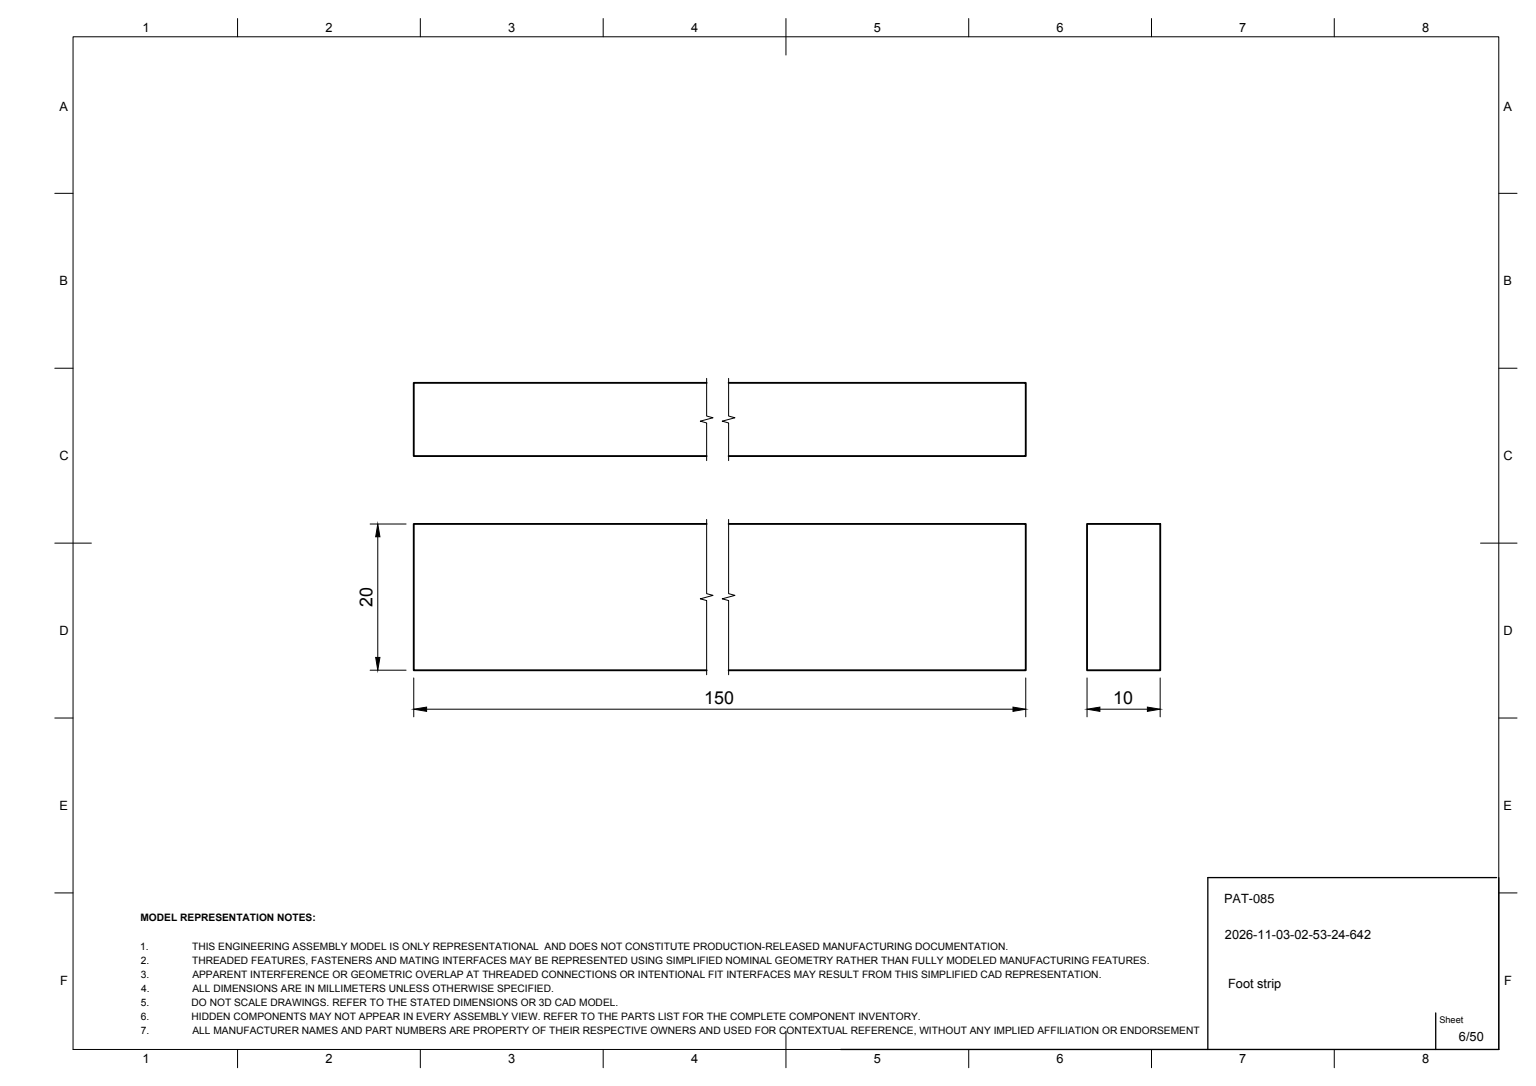
ISO-10303-21;
HEADER;
/* Generated by software containing ST-Developer
 * from STEP Tools, Inc. (www.steptools.com) 
 */

FILE_DESCRIPTION(
/* description */ ('Rack and pinion manual slide'),
/* implementation_level */ '2;1');

FILE_NAME(
/* name */ 'Foot strip.step',
/* time_stamp */ '2026-10-28T03:22:49-07:00',
/* author */ (''),
/* organization */ (''),
/* preprocessor_version */ 'ST-DEVELOPER v20.2',
/* originating_system */ 'Autodesk Translation Framework v15.17.0.0',
/* authorisation */ '');

FILE_SCHEMA (('AUTOMOTIVE_DESIGN { 1 0 10303 214 3 1 1 }'));
ENDSEC;

DATA;
#10=MECHANICAL_DESIGN_GEOMETRIC_PRESENTATION_REPRESENTATION('',(#733),#34851);
#641=SHAPE_REPRESENTATION_RELATIONSHIP('SRR','None',#35076,#687);
#687=ADVANCED_BREP_SHAPE_REPRESENTATION('',(#786),#34801);
#733=STYLED_ITEM('',(#35397),#786);
#786=MANIFOLD_SOLID_BREP('Body1',#13753);
#1050=PLANE('',#14339);
#1051=PLANE('',#14340);
#1052=PLANE('',#14341);
#1053=PLANE('',#14342);
#1054=PLANE('',#14343);
#1055=PLANE('',#14344);
#1545=FACE_OUTER_BOUND('',#2292,.T.);
#1546=FACE_OUTER_BOUND('',#2293,.T.);
#1547=FACE_OUTER_BOUND('',#2294,.T.);
#1548=FACE_OUTER_BOUND('',#2295,.T.);
#1549=FACE_OUTER_BOUND('',#2296,.T.);
#1550=FACE_OUTER_BOUND('',#2297,.T.);
#2292=EDGE_LOOP('',(#9282,#9283,#9284,#9285));
#2293=EDGE_LOOP('',(#9286,#9287,#9288,#9289));
#2294=EDGE_LOOP('',(#9290,#9291,#9292,#9293));
#2295=EDGE_LOOP('',(#9294,#9295,#9296,#9297));
#2296=EDGE_LOOP('',(#9298,#9299,#9300,#9301));
#2297=EDGE_LOOP('',(#9302,#9303,#9304,#9305));
#3240=LINE('',#19514,#4531);
#3241=LINE('',#19516,#4532);
#3242=LINE('',#19518,#4533);
#3243=LINE('',#19519,#4534);
#3244=LINE('',#19522,#4535);
#3245=LINE('',#19524,#4536);
#3246=LINE('',#19525,#4537);
#3247=LINE('',#19528,#4538);
#3248=LINE('',#19530,#4539);
#3249=LINE('',#19531,#4540);
#3250=LINE('',#19533,#4541);
#3251=LINE('',#19534,#4542);
#4531=VECTOR('',#15662,1.);
#4532=VECTOR('',#15663,1.);
#4533=VECTOR('',#15664,1.);
#4534=VECTOR('',#15665,1.);
#4535=VECTOR('',#15668,1.);
#4536=VECTOR('',#15669,1.);
#4537=VECTOR('',#15670,1.);
#4538=VECTOR('',#15673,1.);
#4539=VECTOR('',#15674,1.);
#4540=VECTOR('',#15675,1.);
#4541=VECTOR('',#15678,1.);
#4542=VECTOR('',#15679,1.);
#6240=VERTEX_POINT('',#19512);
#6241=VERTEX_POINT('',#19513);
#6242=VERTEX_POINT('',#19515);
#6243=VERTEX_POINT('',#19517);
#6244=VERTEX_POINT('',#19521);
#6245=VERTEX_POINT('',#19523);
#6246=VERTEX_POINT('',#19527);
#6247=VERTEX_POINT('',#19529);
#7453=EDGE_CURVE('',#6240,#6241,#3240,.T.);
#7454=EDGE_CURVE('',#6241,#6242,#3241,.T.);
#7455=EDGE_CURVE('',#6243,#6242,#3242,.T.);
#7456=EDGE_CURVE('',#6240,#6243,#3243,.T.);
#7457=EDGE_CURVE('',#6244,#6240,#3244,.T.);
#7458=EDGE_CURVE('',#6245,#6243,#3245,.T.);
#7459=EDGE_CURVE('',#6244,#6245,#3246,.T.);
#7460=EDGE_CURVE('',#6246,#6244,#3247,.T.);
#7461=EDGE_CURVE('',#6247,#6245,#3248,.T.);
#7462=EDGE_CURVE('',#6246,#6247,#3249,.T.);
#7463=EDGE_CURVE('',#6241,#6246,#3250,.T.);
#7464=EDGE_CURVE('',#6242,#6247,#3251,.T.);
#9282=ORIENTED_EDGE('',*,*,#7453,.T.);
#9283=ORIENTED_EDGE('',*,*,#7454,.T.);
#9284=ORIENTED_EDGE('',*,*,#7455,.F.);
#9285=ORIENTED_EDGE('',*,*,#7456,.F.);
#9286=ORIENTED_EDGE('',*,*,#7457,.T.);
#9287=ORIENTED_EDGE('',*,*,#7456,.T.);
#9288=ORIENTED_EDGE('',*,*,#7458,.F.);
#9289=ORIENTED_EDGE('',*,*,#7459,.F.);
#9290=ORIENTED_EDGE('',*,*,#7460,.T.);
#9291=ORIENTED_EDGE('',*,*,#7459,.T.);
#9292=ORIENTED_EDGE('',*,*,#7461,.F.);
#9293=ORIENTED_EDGE('',*,*,#7462,.F.);
#9294=ORIENTED_EDGE('',*,*,#7463,.T.);
#9295=ORIENTED_EDGE('',*,*,#7462,.T.);
#9296=ORIENTED_EDGE('',*,*,#7464,.F.);
#9297=ORIENTED_EDGE('',*,*,#7454,.F.);
#9298=ORIENTED_EDGE('',*,*,#7464,.T.);
#9299=ORIENTED_EDGE('',*,*,#7461,.T.);
#9300=ORIENTED_EDGE('',*,*,#7458,.T.);
#9301=ORIENTED_EDGE('',*,*,#7455,.T.);
#9302=ORIENTED_EDGE('',*,*,#7463,.F.);
#9303=ORIENTED_EDGE('',*,*,#7453,.F.);
#9304=ORIENTED_EDGE('',*,*,#7457,.F.);
#9305=ORIENTED_EDGE('',*,*,#7460,.F.);
#13023=ADVANCED_FACE('',(#1545),#1050,.T.);
#13024=ADVANCED_FACE('',(#1546),#1051,.T.);
#13025=ADVANCED_FACE('',(#1547),#1052,.T.);
#13026=ADVANCED_FACE('',(#1548),#1053,.T.);
#13027=ADVANCED_FACE('',(#1549),#1054,.T.);
#13028=ADVANCED_FACE('',(#1550),#1055,.F.);
#13753=CLOSED_SHELL('',(#13023,#13024,#13025,#13026,#13027,#13028));
#14338=AXIS2_PLACEMENT_3D('',#19510,#15658,#15659);
#14339=AXIS2_PLACEMENT_3D('',#19511,#15660,#15661);
#14340=AXIS2_PLACEMENT_3D('',#19520,#15666,#15667);
#14341=AXIS2_PLACEMENT_3D('',#19526,#15671,#15672);
#14342=AXIS2_PLACEMENT_3D('',#19532,#15676,#15677);
#14343=AXIS2_PLACEMENT_3D('',#19535,#15680,#15681);
#14344=AXIS2_PLACEMENT_3D('',#19536,#15682,#15683);
#15658=DIRECTION('axis',(0.,0.,1.));
#15659=DIRECTION('refdir',(1.,0.,0.));
#15660=DIRECTION('center_axis',(0.,1.,0.));
#15661=DIRECTION('ref_axis',(-1.,0.,0.));
#15662=DIRECTION('',(-1.,0.,0.));
#15663=DIRECTION('',(0.,0.,1.));
#15664=DIRECTION('',(-1.,0.,0.));
#15665=DIRECTION('',(0.,0.,1.));
#15666=DIRECTION('center_axis',(1.,0.,0.));
#15667=DIRECTION('ref_axis',(0.,1.,0.));
#15668=DIRECTION('',(0.,1.,0.));
#15669=DIRECTION('',(0.,1.,0.));
#15670=DIRECTION('',(0.,0.,1.));
#15671=DIRECTION('center_axis',(0.,-1.,0.));
#15672=DIRECTION('ref_axis',(1.,0.,0.));
#15673=DIRECTION('',(1.,0.,0.));
#15674=DIRECTION('',(1.,0.,0.));
#15675=DIRECTION('',(0.,0.,1.));
#15676=DIRECTION('center_axis',(-1.,0.,0.));
#15677=DIRECTION('ref_axis',(0.,-1.,0.));
#15678=DIRECTION('',(0.,-1.,0.));
#15679=DIRECTION('',(0.,-1.,0.));
#15680=DIRECTION('center_axis',(0.,0.,1.));
#15681=DIRECTION('ref_axis',(1.,0.,0.));
#15682=DIRECTION('center_axis',(0.,0.,1.));
#15683=DIRECTION('ref_axis',(1.,0.,0.));
#19510=CARTESIAN_POINT('',(0.,0.,0.));
#19511=CARTESIAN_POINT('Origin',(-4.,7.5,-1.));
#19512=CARTESIAN_POINT('',(-4.,7.5,-1.));
#19513=CARTESIAN_POINT('',(-6.,7.5,-1.));
#19514=CARTESIAN_POINT('',(-4.,7.5,-1.));
#19515=CARTESIAN_POINT('',(-6.,7.5,0.));
#19516=CARTESIAN_POINT('',(-6.,7.5,-1.));
#19517=CARTESIAN_POINT('',(-4.,7.5,0.));
#19518=CARTESIAN_POINT('',(-4.,7.5,0.));
#19519=CARTESIAN_POINT('',(-4.,7.5,-1.));
#19520=CARTESIAN_POINT('Origin',(-4.,-7.5,-1.));
#19521=CARTESIAN_POINT('',(-4.,-7.5,-1.));
#19522=CARTESIAN_POINT('',(-4.,-7.5,-1.));
#19523=CARTESIAN_POINT('',(-4.,-7.5,0.));
#19524=CARTESIAN_POINT('',(-4.,-7.5,0.));
#19525=CARTESIAN_POINT('',(-4.,-7.5,-1.));
#19526=CARTESIAN_POINT('Origin',(-6.,-7.5,-1.));
#19527=CARTESIAN_POINT('',(-6.,-7.5,-1.));
#19528=CARTESIAN_POINT('',(-6.,-7.5,-1.));
#19529=CARTESIAN_POINT('',(-6.,-7.5,0.));
#19530=CARTESIAN_POINT('',(-6.,-7.5,0.));
#19531=CARTESIAN_POINT('',(-6.,-7.5,-1.));
#19532=CARTESIAN_POINT('Origin',(-6.,7.5,-1.));
#19533=CARTESIAN_POINT('',(-6.,7.5,-1.));
#19534=CARTESIAN_POINT('',(-6.,7.5,0.));
#19535=CARTESIAN_POINT('Origin',(-5.,0.,0.));
#19536=CARTESIAN_POINT('Origin',(-5.,0.,-1.));
#34747=UNCERTAINTY_MEASURE_WITH_UNIT(LENGTH_MEASURE(0.001),#34852,
'DISTANCE_ACCURACY_VALUE',
'Maximum model space distance between geometric entities at asserted c
onnectivities');
#34797=UNCERTAINTY_MEASURE_WITH_UNIT(LENGTH_MEASURE(0.001),#34852,
'DISTANCE_ACCURACY_VALUE',
'Maximum model space distance between geometric entities at asserted c
onnectivities');
#34801=(
GEOMETRIC_REPRESENTATION_CONTEXT(3)
GLOBAL_UNCERTAINTY_ASSIGNED_CONTEXT((#34747))
GLOBAL_UNIT_ASSIGNED_CONTEXT((#34852,#34854,#34855))
REPRESENTATION_CONTEXT('','3D')
);
#34851=(
GEOMETRIC_REPRESENTATION_CONTEXT(3)
GLOBAL_UNCERTAINTY_ASSIGNED_CONTEXT((#34797))
GLOBAL_UNIT_ASSIGNED_CONTEXT((#34852,#34854,#34855))
REPRESENTATION_CONTEXT('','3D')
);
#34852=(
LENGTH_UNIT()
NAMED_UNIT(*)
SI_UNIT(.CENTI.,.METRE.)
);
#34854=(
NAMED_UNIT(*)
PLANE_ANGLE_UNIT()
SI_UNIT($,.RADIAN.)
);
#34855=(
NAMED_UNIT(*)
SI_UNIT($,.STERADIAN.)
SOLID_ANGLE_UNIT()
);
#34859=SHAPE_DEFINITION_REPRESENTATION(#34912,#35076);
#34912=PRODUCT_DEFINITION_SHAPE('',$,#35130);
#35076=SHAPE_REPRESENTATION('',(#14338),#34801);
#35126=PRODUCT_DEFINITION_CONTEXT('part definition',#35287,'design');
#35130=PRODUCT_DEFINITION('Foot strip','Foot strip',#35183,#35126);
#35183=PRODUCT_DEFINITION_FORMATION('',$,#35292);
#35287=APPLICATION_CONTEXT(
'Core Data for Automotive Mechanical Design Process');
#35288=PRODUCT_CONTEXT('part definition',#35287,'mechanical');
#35292=PRODUCT('Foot strip','Foot strip','Foot strip',(#35288));
#35391=COLOUR_RGB('Light Blue',0.38,0.62,0.78);
#35392=FILL_AREA_STYLE_COLOUR('',#35391);
#35393=FILL_AREA_STYLE('',(#35392));
#35394=SURFACE_STYLE_FILL_AREA(#35393);
#35395=SURFACE_SIDE_STYLE('',(#35394));
#35396=SURFACE_STYLE_USAGE(.BOTH.,#35395);
#35397=PRESENTATION_STYLE_ASSIGNMENT((#35396));
ENDSEC;
END-ISO-10303-21;
